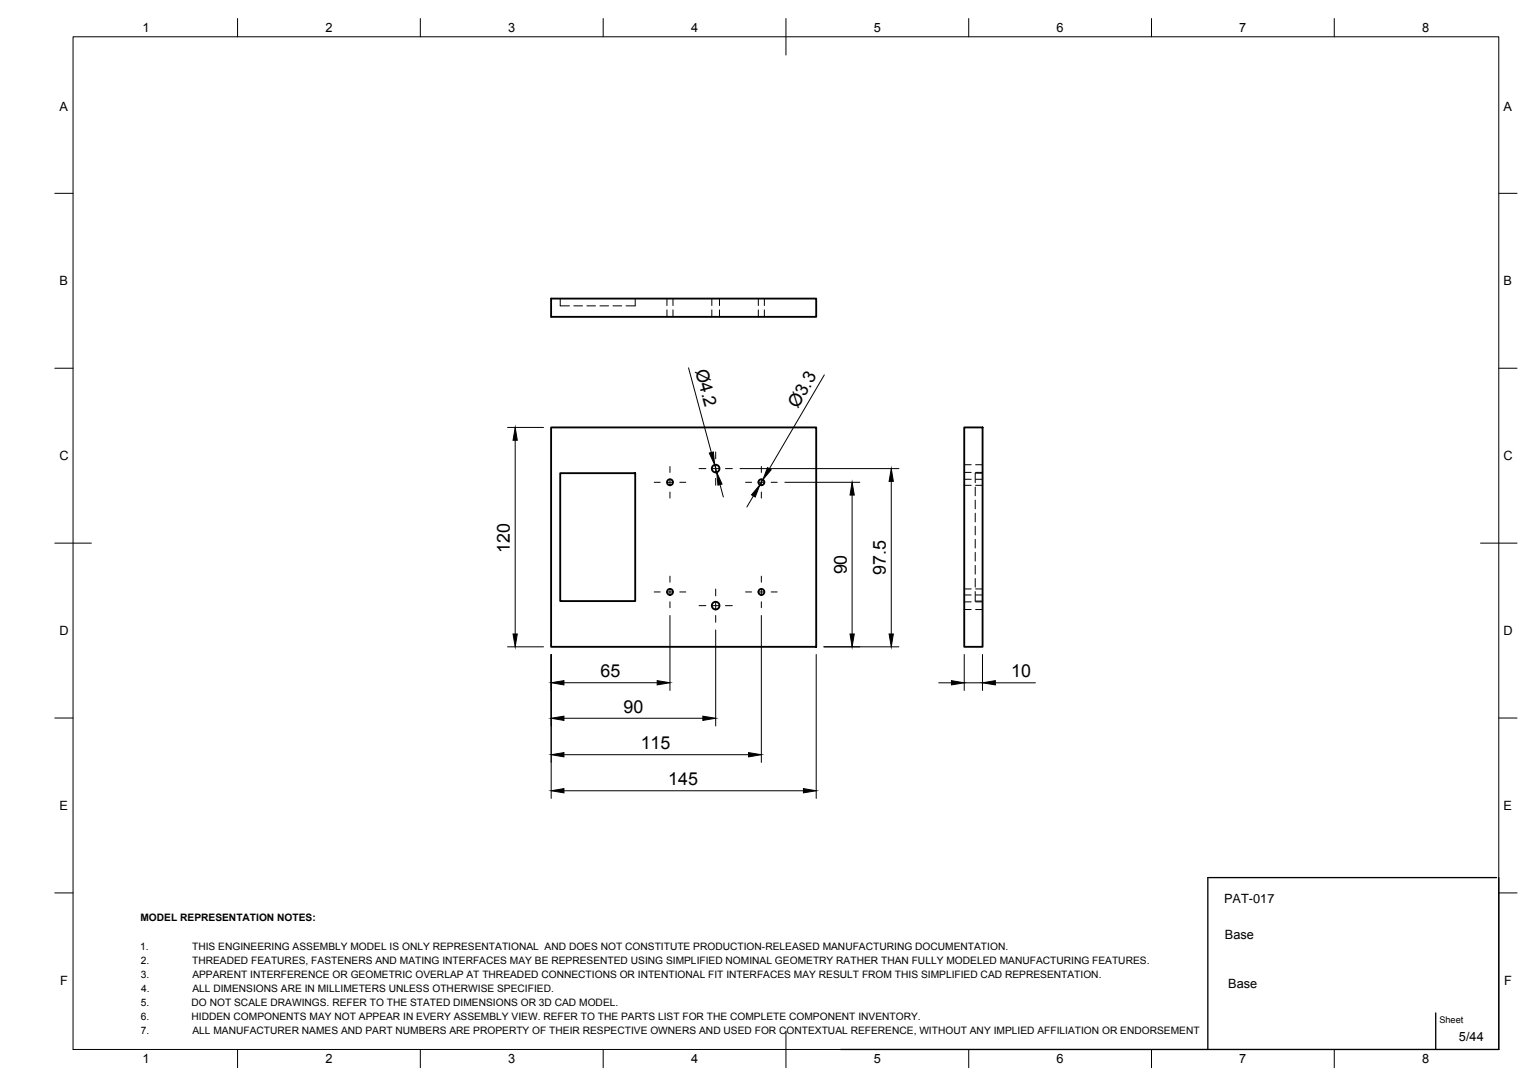
ISO-10303-21;
HEADER;
/* Generated by software containing ST-Developer
 * from STEP Tools, Inc. (www.steptools.com) 
 */

FILE_DESCRIPTION(
/* description */ ('Cam-and-follower valve demonstrator'),
/* implementation_level */ '2;1');

FILE_NAME(
/* name */ 'Base.step',
/* time_stamp */ '2026-10-28T03:25:17-07:00',
/* author */ (''),
/* organization */ (''),
/* preprocessor_version */ 'ST-DEVELOPER v20.2',
/* originating_system */ 'Autodesk Translation Framework v15.17.0.0',
/* authorisation */ '');

FILE_SCHEMA (('AUTOMOTIVE_DESIGN { 1 0 10303 214 3 1 1 }'));
ENDSEC;

DATA;
#10=MECHANICAL_DESIGN_GEOMETRIC_PRESENTATION_REPRESENTATION('',(#412),#12896);
#340=SHAPE_REPRESENTATION_RELATIONSHIP('SRR','None',#13056,#376);
#376=ADVANCED_BREP_SHAPE_REPRESENTATION('',(#455),#12856);
#412=STYLED_ITEM('',(#13309),#455);
#455=MANIFOLD_SOLID_BREP('Body1',#6179);
#495=FACE_BOUND('',#1479,.T.);
#496=FACE_BOUND('',#1480,.T.);
#497=FACE_BOUND('',#1481,.T.);
#498=FACE_BOUND('',#1482,.T.);
#499=FACE_BOUND('',#1483,.T.);
#500=FACE_BOUND('',#1484,.T.);
#501=FACE_BOUND('',#1485,.T.);
#502=FACE_BOUND('',#1487,.T.);
#503=FACE_BOUND('',#1488,.T.);
#504=FACE_BOUND('',#1489,.T.);
#505=FACE_BOUND('',#1490,.T.);
#506=FACE_BOUND('',#1491,.T.);
#507=FACE_BOUND('',#1492,.T.);
#659=CIRCLE('',#6631,0.21);
#660=CIRCLE('',#6632,0.21);
#661=CIRCLE('',#6634,0.21);
#662=CIRCLE('',#6635,0.21);
#663=CIRCLE('',#6637,0.165);
#664=CIRCLE('',#6638,0.165);
#665=CIRCLE('',#6640,0.165);
#666=CIRCLE('',#6641,0.165);
#667=CIRCLE('',#6643,0.165);
#668=CIRCLE('',#6644,0.165);
#669=CIRCLE('',#6646,0.165);
#670=CIRCLE('',#6647,0.165);
#973=CYLINDRICAL_SURFACE('',#6630,0.21);
#974=CYLINDRICAL_SURFACE('',#6633,0.21);
#975=CYLINDRICAL_SURFACE('',#6636,0.165);
#976=CYLINDRICAL_SURFACE('',#6639,0.165);
#977=CYLINDRICAL_SURFACE('',#6642,0.165);
#978=CYLINDRICAL_SURFACE('',#6645,0.165);
#1095=FACE_OUTER_BOUND('',#1463,.T.);
#1096=FACE_OUTER_BOUND('',#1464,.T.);
#1097=FACE_OUTER_BOUND('',#1465,.T.);
#1098=FACE_OUTER_BOUND('',#1466,.T.);
#1099=FACE_OUTER_BOUND('',#1467,.T.);
#1100=FACE_OUTER_BOUND('',#1468,.T.);
#1101=FACE_OUTER_BOUND('',#1469,.T.);
#1102=FACE_OUTER_BOUND('',#1470,.T.);
#1103=FACE_OUTER_BOUND('',#1471,.T.);
#1104=FACE_OUTER_BOUND('',#1472,.T.);
#1105=FACE_OUTER_BOUND('',#1473,.T.);
#1106=FACE_OUTER_BOUND('',#1474,.T.);
#1107=FACE_OUTER_BOUND('',#1475,.T.);
#1108=FACE_OUTER_BOUND('',#1476,.T.);
#1109=FACE_OUTER_BOUND('',#1477,.T.);
#1110=FACE_OUTER_BOUND('',#1478,.T.);
#1111=FACE_OUTER_BOUND('',#1486,.T.);
#1463=EDGE_LOOP('',(#4095,#4096,#4097,#4098));
#1464=EDGE_LOOP('',(#4099,#4100,#4101,#4102));
#1465=EDGE_LOOP('',(#4103,#4104,#4105,#4106));
#1466=EDGE_LOOP('',(#4107,#4108,#4109,#4110));
#1467=EDGE_LOOP('',(#4111,#4112,#4113,#4114));
#1468=EDGE_LOOP('',(#4115,#4116,#4117,#4118));
#1469=EDGE_LOOP('',(#4119,#4120,#4121,#4122));
#1470=EDGE_LOOP('',(#4123,#4124,#4125,#4126));
#1471=EDGE_LOOP('',(#4127,#4128,#4129,#4130));
#1472=EDGE_LOOP('',(#4131,#4132,#4133,#4134));
#1473=EDGE_LOOP('',(#4135,#4136,#4137,#4138));
#1474=EDGE_LOOP('',(#4139,#4140,#4141,#4142));
#1475=EDGE_LOOP('',(#4143,#4144,#4145,#4146));
#1476=EDGE_LOOP('',(#4147,#4148,#4149,#4150));
#1477=EDGE_LOOP('',(#4151,#4152,#4153,#4154));
#1478=EDGE_LOOP('',(#4155,#4156,#4157,#4158));
#1479=EDGE_LOOP('',(#4159,#4160,#4161,#4162));
#1480=EDGE_LOOP('',(#4163));
#1481=EDGE_LOOP('',(#4164));
#1482=EDGE_LOOP('',(#4165));
#1483=EDGE_LOOP('',(#4166));
#1484=EDGE_LOOP('',(#4167));
#1485=EDGE_LOOP('',(#4168));
#1486=EDGE_LOOP('',(#4169,#4170,#4171,#4172));
#1487=EDGE_LOOP('',(#4173));
#1488=EDGE_LOOP('',(#4174));
#1489=EDGE_LOOP('',(#4175));
#1490=EDGE_LOOP('',(#4176));
#1491=EDGE_LOOP('',(#4177));
#1492=EDGE_LOOP('',(#4178));
#1995=LINE('',#9426,#2417);
#1996=LINE('',#9428,#2418);
#1997=LINE('',#9430,#2419);
#1998=LINE('',#9431,#2420);
#1999=LINE('',#9434,#2421);
#2000=LINE('',#9436,#2422);
#2001=LINE('',#9437,#2423);
#2002=LINE('',#9440,#2424);
#2003=LINE('',#9442,#2425);
#2004=LINE('',#9443,#2426);
#2005=LINE('',#9445,#2427);
#2006=LINE('',#9446,#2428);
#2007=LINE('',#9452,#2429);
#2008=LINE('',#9458,#2430);
#2009=LINE('',#9464,#2431);
#2010=LINE('',#9470,#2432);
#2011=LINE('',#9476,#2433);
#2012=LINE('',#9482,#2434);
#2013=LINE('',#9487,#2435);
#2014=LINE('',#9489,#2436);
#2015=LINE('',#9491,#2437);
#2016=LINE('',#9492,#2438);
#2017=LINE('',#9495,#2439);
#2018=LINE('',#9497,#2440);
#2019=LINE('',#9498,#2441);
#2020=LINE('',#9501,#2442);
#2021=LINE('',#9503,#2443);
#2022=LINE('',#9504,#2444);
#2023=LINE('',#9506,#2445);
#2024=LINE('',#9507,#2446);
#2417=VECTOR('',#7422,1.);
#2418=VECTOR('',#7423,1.);
#2419=VECTOR('',#7424,1.);
#2420=VECTOR('',#7425,1.);
#2421=VECTOR('',#7428,1.);
#2422=VECTOR('',#7429,1.);
#2423=VECTOR('',#7430,1.);
#2424=VECTOR('',#7433,1.);
#2425=VECTOR('',#7434,1.);
#2426=VECTOR('',#7435,1.);
#2427=VECTOR('',#7438,1.);
#2428=VECTOR('',#7439,1.);
#2429=VECTOR('',#7446,0.21);
#2430=VECTOR('',#7453,0.21);
#2431=VECTOR('',#7460,0.165);
#2432=VECTOR('',#7467,0.165);
#2433=VECTOR('',#7474,0.165);
#2434=VECTOR('',#7481,0.165);
#2435=VECTOR('',#7486,1.);
#2436=VECTOR('',#7487,1.);
#2437=VECTOR('',#7488,1.);
#2438=VECTOR('',#7489,1.);
#2439=VECTOR('',#7492,1.);
#2440=VECTOR('',#7493,1.);
#2441=VECTOR('',#7494,1.);
#2442=VECTOR('',#7497,1.);
#2443=VECTOR('',#7498,1.);
#2444=VECTOR('',#7499,1.);
#2445=VECTOR('',#7502,1.);
#2446=VECTOR('',#7503,1.);
#2839=VERTEX_POINT('',#9424);
#2840=VERTEX_POINT('',#9425);
#2841=VERTEX_POINT('',#9427);
#2842=VERTEX_POINT('',#9429);
#2843=VERTEX_POINT('',#9433);
#2844=VERTEX_POINT('',#9435);
#2845=VERTEX_POINT('',#9439);
#2846=VERTEX_POINT('',#9441);
#2847=VERTEX_POINT('',#9449);
#2848=VERTEX_POINT('',#9451);
#2849=VERTEX_POINT('',#9455);
#2850=VERTEX_POINT('',#9457);
#2851=VERTEX_POINT('',#9461);
#2852=VERTEX_POINT('',#9463);
#2853=VERTEX_POINT('',#9467);
#2854=VERTEX_POINT('',#9469);
#2855=VERTEX_POINT('',#9473);
#2856=VERTEX_POINT('',#9475);
#2857=VERTEX_POINT('',#9479);
#2858=VERTEX_POINT('',#9481);
#2859=VERTEX_POINT('',#9485);
#2860=VERTEX_POINT('',#9486);
#2861=VERTEX_POINT('',#9488);
#2862=VERTEX_POINT('',#9490);
#2863=VERTEX_POINT('',#9494);
#2864=VERTEX_POINT('',#9496);
#2865=VERTEX_POINT('',#9500);
#2866=VERTEX_POINT('',#9502);
#3344=EDGE_CURVE('',#2839,#2840,#1995,.T.);
#3345=EDGE_CURVE('',#2841,#2839,#1996,.T.);
#3346=EDGE_CURVE('',#2842,#2841,#1997,.T.);
#3347=EDGE_CURVE('',#2842,#2840,#1998,.T.);
#3348=EDGE_CURVE('',#2840,#2843,#1999,.T.);
#3349=EDGE_CURVE('',#2844,#2842,#2000,.T.);
#3350=EDGE_CURVE('',#2844,#2843,#2001,.T.);
#3351=EDGE_CURVE('',#2843,#2845,#2002,.T.);
#3352=EDGE_CURVE('',#2846,#2844,#2003,.T.);
#3353=EDGE_CURVE('',#2846,#2845,#2004,.T.);
#3354=EDGE_CURVE('',#2845,#2839,#2005,.T.);
#3355=EDGE_CURVE('',#2841,#2846,#2006,.T.);
#3356=EDGE_CURVE('',#2847,#2847,#659,.T.);
#3357=EDGE_CURVE('',#2847,#2848,#2007,.T.);
#3358=EDGE_CURVE('',#2848,#2848,#660,.T.);
#3359=EDGE_CURVE('',#2849,#2849,#661,.T.);
#3360=EDGE_CURVE('',#2849,#2850,#2008,.T.);
#3361=EDGE_CURVE('',#2850,#2850,#662,.T.);
#3362=EDGE_CURVE('',#2851,#2851,#663,.T.);
#3363=EDGE_CURVE('',#2851,#2852,#2009,.T.);
#3364=EDGE_CURVE('',#2852,#2852,#664,.T.);
#3365=EDGE_CURVE('',#2853,#2853,#665,.T.);
#3366=EDGE_CURVE('',#2853,#2854,#2010,.T.);
#3367=EDGE_CURVE('',#2854,#2854,#666,.T.);
#3368=EDGE_CURVE('',#2855,#2855,#667,.T.);
#3369=EDGE_CURVE('',#2855,#2856,#2011,.T.);
#3370=EDGE_CURVE('',#2856,#2856,#668,.T.);
#3371=EDGE_CURVE('',#2857,#2857,#669,.T.);
#3372=EDGE_CURVE('',#2857,#2858,#2012,.T.);
#3373=EDGE_CURVE('',#2858,#2858,#670,.T.);
#3374=EDGE_CURVE('',#2859,#2860,#2013,.T.);
#3375=EDGE_CURVE('',#2860,#2861,#2014,.T.);
#3376=EDGE_CURVE('',#2862,#2861,#2015,.T.);
#3377=EDGE_CURVE('',#2859,#2862,#2016,.T.);
#3378=EDGE_CURVE('',#2863,#2859,#2017,.T.);
#3379=EDGE_CURVE('',#2864,#2862,#2018,.T.);
#3380=EDGE_CURVE('',#2863,#2864,#2019,.T.);
#3381=EDGE_CURVE('',#2865,#2863,#2020,.T.);
#3382=EDGE_CURVE('',#2866,#2864,#2021,.T.);
#3383=EDGE_CURVE('',#2865,#2866,#2022,.T.);
#3384=EDGE_CURVE('',#2860,#2865,#2023,.T.);
#3385=EDGE_CURVE('',#2861,#2866,#2024,.T.);
#4095=ORIENTED_EDGE('',*,*,#3344,.F.);
#4096=ORIENTED_EDGE('',*,*,#3345,.F.);
#4097=ORIENTED_EDGE('',*,*,#3346,.F.);
#4098=ORIENTED_EDGE('',*,*,#3347,.T.);
#4099=ORIENTED_EDGE('',*,*,#3348,.F.);
#4100=ORIENTED_EDGE('',*,*,#3347,.F.);
#4101=ORIENTED_EDGE('',*,*,#3349,.F.);
#4102=ORIENTED_EDGE('',*,*,#3350,.T.);
#4103=ORIENTED_EDGE('',*,*,#3351,.F.);
#4104=ORIENTED_EDGE('',*,*,#3350,.F.);
#4105=ORIENTED_EDGE('',*,*,#3352,.F.);
#4106=ORIENTED_EDGE('',*,*,#3353,.T.);
#4107=ORIENTED_EDGE('',*,*,#3354,.F.);
#4108=ORIENTED_EDGE('',*,*,#3353,.F.);
#4109=ORIENTED_EDGE('',*,*,#3355,.F.);
#4110=ORIENTED_EDGE('',*,*,#3345,.T.);
#4111=ORIENTED_EDGE('',*,*,#3349,.T.);
#4112=ORIENTED_EDGE('',*,*,#3346,.T.);
#4113=ORIENTED_EDGE('',*,*,#3355,.T.);
#4114=ORIENTED_EDGE('',*,*,#3352,.T.);
#4115=ORIENTED_EDGE('',*,*,#3356,.F.);
#4116=ORIENTED_EDGE('',*,*,#3357,.T.);
#4117=ORIENTED_EDGE('',*,*,#3358,.F.);
#4118=ORIENTED_EDGE('',*,*,#3357,.F.);
#4119=ORIENTED_EDGE('',*,*,#3359,.F.);
#4120=ORIENTED_EDGE('',*,*,#3360,.T.);
#4121=ORIENTED_EDGE('',*,*,#3361,.F.);
#4122=ORIENTED_EDGE('',*,*,#3360,.F.);
#4123=ORIENTED_EDGE('',*,*,#3362,.F.);
#4124=ORIENTED_EDGE('',*,*,#3363,.T.);
#4125=ORIENTED_EDGE('',*,*,#3364,.F.);
#4126=ORIENTED_EDGE('',*,*,#3363,.F.);
#4127=ORIENTED_EDGE('',*,*,#3365,.F.);
#4128=ORIENTED_EDGE('',*,*,#3366,.T.);
#4129=ORIENTED_EDGE('',*,*,#3367,.F.);
#4130=ORIENTED_EDGE('',*,*,#3366,.F.);
#4131=ORIENTED_EDGE('',*,*,#3368,.F.);
#4132=ORIENTED_EDGE('',*,*,#3369,.T.);
#4133=ORIENTED_EDGE('',*,*,#3370,.F.);
#4134=ORIENTED_EDGE('',*,*,#3369,.F.);
#4135=ORIENTED_EDGE('',*,*,#3371,.F.);
#4136=ORIENTED_EDGE('',*,*,#3372,.T.);
#4137=ORIENTED_EDGE('',*,*,#3373,.F.);
#4138=ORIENTED_EDGE('',*,*,#3372,.F.);
#4139=ORIENTED_EDGE('',*,*,#3374,.T.);
#4140=ORIENTED_EDGE('',*,*,#3375,.T.);
#4141=ORIENTED_EDGE('',*,*,#3376,.F.);
#4142=ORIENTED_EDGE('',*,*,#3377,.F.);
#4143=ORIENTED_EDGE('',*,*,#3378,.T.);
#4144=ORIENTED_EDGE('',*,*,#3377,.T.);
#4145=ORIENTED_EDGE('',*,*,#3379,.F.);
#4146=ORIENTED_EDGE('',*,*,#3380,.F.);
#4147=ORIENTED_EDGE('',*,*,#3381,.T.);
#4148=ORIENTED_EDGE('',*,*,#3380,.T.);
#4149=ORIENTED_EDGE('',*,*,#3382,.F.);
#4150=ORIENTED_EDGE('',*,*,#3383,.F.);
#4151=ORIENTED_EDGE('',*,*,#3384,.T.);
#4152=ORIENTED_EDGE('',*,*,#3383,.T.);
#4153=ORIENTED_EDGE('',*,*,#3385,.F.);
#4154=ORIENTED_EDGE('',*,*,#3375,.F.);
#4155=ORIENTED_EDGE('',*,*,#3385,.T.);
#4156=ORIENTED_EDGE('',*,*,#3382,.T.);
#4157=ORIENTED_EDGE('',*,*,#3379,.T.);
#4158=ORIENTED_EDGE('',*,*,#3376,.T.);
#4159=ORIENTED_EDGE('',*,*,#3351,.T.);
#4160=ORIENTED_EDGE('',*,*,#3354,.T.);
#4161=ORIENTED_EDGE('',*,*,#3344,.T.);
#4162=ORIENTED_EDGE('',*,*,#3348,.T.);
#4163=ORIENTED_EDGE('',*,*,#3358,.T.);
#4164=ORIENTED_EDGE('',*,*,#3361,.T.);
#4165=ORIENTED_EDGE('',*,*,#3364,.T.);
#4166=ORIENTED_EDGE('',*,*,#3367,.T.);
#4167=ORIENTED_EDGE('',*,*,#3370,.T.);
#4168=ORIENTED_EDGE('',*,*,#3373,.T.);
#4169=ORIENTED_EDGE('',*,*,#3384,.F.);
#4170=ORIENTED_EDGE('',*,*,#3374,.F.);
#4171=ORIENTED_EDGE('',*,*,#3378,.F.);
#4172=ORIENTED_EDGE('',*,*,#3381,.F.);
#4173=ORIENTED_EDGE('',*,*,#3356,.T.);
#4174=ORIENTED_EDGE('',*,*,#3359,.T.);
#4175=ORIENTED_EDGE('',*,*,#3362,.T.);
#4176=ORIENTED_EDGE('',*,*,#3365,.T.);
#4177=ORIENTED_EDGE('',*,*,#3368,.T.);
#4178=ORIENTED_EDGE('',*,*,#3371,.T.);
#5597=PLANE('',#6625);
#5598=PLANE('',#6626);
#5599=PLANE('',#6627);
#5600=PLANE('',#6628);
#5601=PLANE('',#6629);
#5602=PLANE('',#6648);
#5603=PLANE('',#6649);
#5604=PLANE('',#6650);
#5605=PLANE('',#6651);
#5606=PLANE('',#6652);
#5607=PLANE('',#6653);
#5811=ADVANCED_FACE('',(#1095),#5597,.F.);
#5812=ADVANCED_FACE('',(#1096),#5598,.F.);
#5813=ADVANCED_FACE('',(#1097),#5599,.F.);
#5814=ADVANCED_FACE('',(#1098),#5600,.F.);
#5815=ADVANCED_FACE('',(#1099),#5601,.T.);
#5816=ADVANCED_FACE('',(#1100),#973,.F.);
#5817=ADVANCED_FACE('',(#1101),#974,.F.);
#5818=ADVANCED_FACE('',(#1102),#975,.F.);
#5819=ADVANCED_FACE('',(#1103),#976,.F.);
#5820=ADVANCED_FACE('',(#1104),#977,.F.);
#5821=ADVANCED_FACE('',(#1105),#978,.F.);
#5822=ADVANCED_FACE('',(#1106),#5602,.T.);
#5823=ADVANCED_FACE('',(#1107),#5603,.T.);
#5824=ADVANCED_FACE('',(#1108),#5604,.T.);
#5825=ADVANCED_FACE('',(#1109),#5605,.T.);
#5826=ADVANCED_FACE('',(#1110,#495,#496,#497,#498,#499,#500,#501),#5606,
 .T.);
#5827=ADVANCED_FACE('',(#1111,#502,#503,#504,#505,#506,#507),#5607,.F.);
#6179=CLOSED_SHELL('',(#5811,#5812,#5813,#5814,#5815,#5816,#5817,#5818,
#5819,#5820,#5821,#5822,#5823,#5824,#5825,#5826,#5827));
#6624=AXIS2_PLACEMENT_3D('',#9422,#7418,#7419);
#6625=AXIS2_PLACEMENT_3D('',#9423,#7420,#7421);
#6626=AXIS2_PLACEMENT_3D('',#9432,#7426,#7427);
#6627=AXIS2_PLACEMENT_3D('',#9438,#7431,#7432);
#6628=AXIS2_PLACEMENT_3D('',#9444,#7436,#7437);
#6629=AXIS2_PLACEMENT_3D('',#9447,#7440,#7441);
#6630=AXIS2_PLACEMENT_3D('',#9448,#7442,#7443);
#6631=AXIS2_PLACEMENT_3D('',#9450,#7444,#7445);
#6632=AXIS2_PLACEMENT_3D('',#9453,#7447,#7448);
#6633=AXIS2_PLACEMENT_3D('',#9454,#7449,#7450);
#6634=AXIS2_PLACEMENT_3D('',#9456,#7451,#7452);
#6635=AXIS2_PLACEMENT_3D('',#9459,#7454,#7455);
#6636=AXIS2_PLACEMENT_3D('',#9460,#7456,#7457);
#6637=AXIS2_PLACEMENT_3D('',#9462,#7458,#7459);
#6638=AXIS2_PLACEMENT_3D('',#9465,#7461,#7462);
#6639=AXIS2_PLACEMENT_3D('',#9466,#7463,#7464);
#6640=AXIS2_PLACEMENT_3D('',#9468,#7465,#7466);
#6641=AXIS2_PLACEMENT_3D('',#9471,#7468,#7469);
#6642=AXIS2_PLACEMENT_3D('',#9472,#7470,#7471);
#6643=AXIS2_PLACEMENT_3D('',#9474,#7472,#7473);
#6644=AXIS2_PLACEMENT_3D('',#9477,#7475,#7476);
#6645=AXIS2_PLACEMENT_3D('',#9478,#7477,#7478);
#6646=AXIS2_PLACEMENT_3D('',#9480,#7479,#7480);
#6647=AXIS2_PLACEMENT_3D('',#9483,#7482,#7483);
#6648=AXIS2_PLACEMENT_3D('',#9484,#7484,#7485);
#6649=AXIS2_PLACEMENT_3D('',#9493,#7490,#7491);
#6650=AXIS2_PLACEMENT_3D('',#9499,#7495,#7496);
#6651=AXIS2_PLACEMENT_3D('',#9505,#7500,#7501);
#6652=AXIS2_PLACEMENT_3D('',#9508,#7504,#7505);
#6653=AXIS2_PLACEMENT_3D('',#9509,#7506,#7507);
#7418=DIRECTION('axis',(0.,0.,1.));
#7419=DIRECTION('refdir',(1.,0.,0.));
#7420=DIRECTION('center_axis',(0.,-1.,0.));
#7421=DIRECTION('ref_axis',(1.,0.,0.));
#7422=DIRECTION('',(-1.,0.,0.));
#7423=DIRECTION('',(0.,0.,1.));
#7424=DIRECTION('',(1.,0.,0.));
#7425=DIRECTION('',(0.,0.,1.));
#7426=DIRECTION('center_axis',(-1.,0.,0.));
#7427=DIRECTION('ref_axis',(0.,-1.,0.));
#7428=DIRECTION('',(0.,1.,0.));
#7429=DIRECTION('',(0.,-1.,0.));
#7430=DIRECTION('',(0.,0.,1.));
#7431=DIRECTION('center_axis',(0.,1.,0.));
#7432=DIRECTION('ref_axis',(-1.,0.,0.));
#7433=DIRECTION('',(1.,0.,0.));
#7434=DIRECTION('',(-1.,0.,0.));
#7435=DIRECTION('',(0.,0.,1.));
#7436=DIRECTION('center_axis',(1.,0.,0.));
#7437=DIRECTION('ref_axis',(0.,1.,0.));
#7438=DIRECTION('',(0.,-1.,0.));
#7439=DIRECTION('',(0.,1.,0.));
#7440=DIRECTION('center_axis',(0.,0.,1.));
#7441=DIRECTION('ref_axis',(1.,0.,0.));
#7442=DIRECTION('center_axis',(0.,0.,1.));
#7443=DIRECTION('ref_axis',(1.,0.,0.));
#7444=DIRECTION('center_axis',(0.,0.,1.));
#7445=DIRECTION('ref_axis',(1.,0.,0.));
#7446=DIRECTION('',(0.,0.,1.));
#7447=DIRECTION('center_axis',(0.,0.,-1.));
#7448=DIRECTION('ref_axis',(1.,0.,0.));
#7449=DIRECTION('center_axis',(0.,0.,1.));
#7450=DIRECTION('ref_axis',(1.,0.,0.));
#7451=DIRECTION('center_axis',(0.,0.,1.));
#7452=DIRECTION('ref_axis',(1.,0.,0.));
#7453=DIRECTION('',(0.,0.,1.));
#7454=DIRECTION('center_axis',(0.,0.,-1.));
#7455=DIRECTION('ref_axis',(1.,0.,0.));
#7456=DIRECTION('center_axis',(0.,0.,1.));
#7457=DIRECTION('ref_axis',(1.,0.,0.));
#7458=DIRECTION('center_axis',(0.,0.,1.));
#7459=DIRECTION('ref_axis',(1.,0.,0.));
#7460=DIRECTION('',(0.,0.,1.));
#7461=DIRECTION('center_axis',(0.,0.,-1.));
#7462=DIRECTION('ref_axis',(1.,0.,0.));
#7463=DIRECTION('center_axis',(0.,0.,1.));
#7464=DIRECTION('ref_axis',(1.,0.,0.));
#7465=DIRECTION('center_axis',(0.,0.,1.));
#7466=DIRECTION('ref_axis',(1.,0.,0.));
#7467=DIRECTION('',(0.,0.,1.));
#7468=DIRECTION('center_axis',(0.,0.,-1.));
#7469=DIRECTION('ref_axis',(1.,0.,0.));
#7470=DIRECTION('center_axis',(0.,0.,1.));
#7471=DIRECTION('ref_axis',(1.,0.,0.));
#7472=DIRECTION('center_axis',(0.,0.,1.));
#7473=DIRECTION('ref_axis',(1.,0.,0.));
#7474=DIRECTION('',(0.,0.,1.));
#7475=DIRECTION('center_axis',(0.,0.,-1.));
#7476=DIRECTION('ref_axis',(1.,0.,0.));
#7477=DIRECTION('center_axis',(0.,0.,1.));
#7478=DIRECTION('ref_axis',(1.,0.,0.));
#7479=DIRECTION('center_axis',(0.,0.,1.));
#7480=DIRECTION('ref_axis',(1.,0.,0.));
#7481=DIRECTION('',(0.,0.,1.));
#7482=DIRECTION('center_axis',(0.,0.,-1.));
#7483=DIRECTION('ref_axis',(1.,0.,0.));
#7484=DIRECTION('center_axis',(0.,1.,0.));
#7485=DIRECTION('ref_axis',(-1.,0.,0.));
#7486=DIRECTION('',(-1.,0.,0.));
#7487=DIRECTION('',(0.,0.,1.));
#7488=DIRECTION('',(-1.,0.,0.));
#7489=DIRECTION('',(0.,0.,1.));
#7490=DIRECTION('center_axis',(1.,0.,0.));
#7491=DIRECTION('ref_axis',(0.,1.,0.));
#7492=DIRECTION('',(0.,1.,0.));
#7493=DIRECTION('',(0.,1.,0.));
#7494=DIRECTION('',(0.,0.,1.));
#7495=DIRECTION('center_axis',(0.,-1.,0.));
#7496=DIRECTION('ref_axis',(1.,0.,0.));
#7497=DIRECTION('',(1.,0.,0.));
#7498=DIRECTION('',(1.,0.,0.));
#7499=DIRECTION('',(0.,0.,1.));
#7500=DIRECTION('center_axis',(-1.,0.,0.));
#7501=DIRECTION('ref_axis',(0.,-1.,0.));
#7502=DIRECTION('',(0.,-1.,0.));
#7503=DIRECTION('',(0.,-1.,0.));
#7504=DIRECTION('center_axis',(0.,0.,1.));
#7505=DIRECTION('ref_axis',(1.,0.,0.));
#7506=DIRECTION('center_axis',(0.,0.,1.));
#7507=DIRECTION('ref_axis',(1.,0.,0.));
#9422=CARTESIAN_POINT('',(0.,0.,0.));
#9423=CARTESIAN_POINT('Origin',(-3.5,4.4,0.6));
#9424=CARTESIAN_POINT('',(3.5,4.4,1.));
#9425=CARTESIAN_POINT('',(-3.5,4.4,1.));
#9426=CARTESIAN_POINT('',(-1.75,4.4,1.));
#9427=CARTESIAN_POINT('',(3.5,4.4,0.6));
#9428=CARTESIAN_POINT('',(3.5,4.4,0.6));
#9429=CARTESIAN_POINT('',(-3.5,4.4,0.6));
#9430=CARTESIAN_POINT('',(-3.5,4.4,0.6));
#9431=CARTESIAN_POINT('',(-3.5,4.4,0.6));
#9432=CARTESIAN_POINT('Origin',(-3.5,8.5,0.6));
#9433=CARTESIAN_POINT('',(-3.5,8.5,1.));
#9434=CARTESIAN_POINT('',(-3.5,5.125,1.));
#9435=CARTESIAN_POINT('',(-3.5,8.5,0.6));
#9436=CARTESIAN_POINT('',(-3.5,8.5,0.6));
#9437=CARTESIAN_POINT('',(-3.5,8.5,0.6));
#9438=CARTESIAN_POINT('Origin',(3.5,8.5,0.6));
#9439=CARTESIAN_POINT('',(3.5,8.5,1.));
#9440=CARTESIAN_POINT('',(1.75,8.5,1.));
#9441=CARTESIAN_POINT('',(3.5,8.5,0.6));
#9442=CARTESIAN_POINT('',(3.5,8.5,0.6));
#9443=CARTESIAN_POINT('',(3.5,8.5,0.6));
#9444=CARTESIAN_POINT('Origin',(3.5,4.4,0.6));
#9445=CARTESIAN_POINT('',(3.5,3.075,1.));
#9446=CARTESIAN_POINT('',(3.5,4.4,0.6));
#9447=CARTESIAN_POINT('Origin',(0.,6.45,0.6));
#9448=CARTESIAN_POINT('Origin',(3.75,0.,-0.1));
#9449=CARTESIAN_POINT('',(3.54,-2.57175827820944E-17,0.));
#9450=CARTESIAN_POINT('Origin',(3.75,0.,0.));
#9451=CARTESIAN_POINT('',(3.54,2.57175827820944E-17,1.));
#9452=CARTESIAN_POINT('',(3.54,-2.57175827820944E-17,-0.1));
#9453=CARTESIAN_POINT('Origin',(3.75,0.,1.));
#9454=CARTESIAN_POINT('Origin',(-3.75,0.,-0.1));
#9455=CARTESIAN_POINT('',(-3.96,-2.57175827820944E-17,0.));
#9456=CARTESIAN_POINT('Origin',(-3.75,0.,0.));
#9457=CARTESIAN_POINT('',(-3.96,2.57175827820944E-17,1.));
#9458=CARTESIAN_POINT('',(-3.96,-2.57175827820944E-17,-0.1));
#9459=CARTESIAN_POINT('Origin',(-3.75,0.,1.));
#9460=CARTESIAN_POINT('Origin',(-3.,2.5,-0.1));
#9461=CARTESIAN_POINT('',(-3.165,2.5,0.));
#9462=CARTESIAN_POINT('Origin',(-3.,2.5,0.));
#9463=CARTESIAN_POINT('',(-3.165,2.5,1.));
#9464=CARTESIAN_POINT('',(-3.165,2.5,-0.1));
#9465=CARTESIAN_POINT('Origin',(-3.,2.5,1.));
#9466=CARTESIAN_POINT('Origin',(3.,2.5,-0.1));
#9467=CARTESIAN_POINT('',(2.835,2.5,0.));
#9468=CARTESIAN_POINT('Origin',(3.,2.5,0.));
#9469=CARTESIAN_POINT('',(2.835,2.5,1.));
#9470=CARTESIAN_POINT('',(2.835,2.5,-0.1));
#9471=CARTESIAN_POINT('Origin',(3.,2.5,1.));
#9472=CARTESIAN_POINT('Origin',(-3.,-2.5,-0.1));
#9473=CARTESIAN_POINT('',(-3.165,-2.5,0.));
#9474=CARTESIAN_POINT('Origin',(-3.,-2.5,0.));
#9475=CARTESIAN_POINT('',(-3.165,-2.5,1.));
#9476=CARTESIAN_POINT('',(-3.165,-2.5,-0.1));
#9477=CARTESIAN_POINT('Origin',(-3.,-2.5,1.));
#9478=CARTESIAN_POINT('Origin',(3.,-2.5,-0.1));
#9479=CARTESIAN_POINT('',(2.835,-2.5,0.));
#9480=CARTESIAN_POINT('Origin',(3.,-2.5,0.));
#9481=CARTESIAN_POINT('',(2.835,-2.5,1.));
#9482=CARTESIAN_POINT('',(2.835,-2.5,-0.1));
#9483=CARTESIAN_POINT('Origin',(3.,-2.5,1.));
#9484=CARTESIAN_POINT('Origin',(6.,9.,0.));
#9485=CARTESIAN_POINT('',(6.,9.,0.));
#9486=CARTESIAN_POINT('',(-6.,9.,0.));
#9487=CARTESIAN_POINT('',(6.,9.,0.));
#9488=CARTESIAN_POINT('',(-6.,9.,1.));
#9489=CARTESIAN_POINT('',(-6.,9.,0.));
#9490=CARTESIAN_POINT('',(6.,9.,1.));
#9491=CARTESIAN_POINT('',(6.,9.,1.));
#9492=CARTESIAN_POINT('',(6.,9.,0.));
#9493=CARTESIAN_POINT('Origin',(6.,-5.5,0.));
#9494=CARTESIAN_POINT('',(6.,-5.5,0.));
#9495=CARTESIAN_POINT('',(6.,-5.5,0.));
#9496=CARTESIAN_POINT('',(6.,-5.5,1.));
#9497=CARTESIAN_POINT('',(6.,-5.5,1.));
#9498=CARTESIAN_POINT('',(6.,-5.5,0.));
#9499=CARTESIAN_POINT('Origin',(-6.,-5.5,0.));
#9500=CARTESIAN_POINT('',(-6.,-5.5,0.));
#9501=CARTESIAN_POINT('',(-6.,-5.5,0.));
#9502=CARTESIAN_POINT('',(-6.,-5.5,1.));
#9503=CARTESIAN_POINT('',(-6.,-5.5,1.));
#9504=CARTESIAN_POINT('',(-6.,-5.5,0.));
#9505=CARTESIAN_POINT('Origin',(-6.,9.,0.));
#9506=CARTESIAN_POINT('',(-6.,9.,0.));
#9507=CARTESIAN_POINT('',(-6.,9.,1.));
#9508=CARTESIAN_POINT('Origin',(0.,1.75,1.));
#9509=CARTESIAN_POINT('Origin',(0.,1.75,0.));
#12813=UNCERTAINTY_MEASURE_WITH_UNIT(LENGTH_MEASURE(0.001),#12897,
'DISTANCE_ACCURACY_VALUE',
'Maximum model space distance between geometric entities at asserted c
onnectivities');
#12853=UNCERTAINTY_MEASURE_WITH_UNIT(LENGTH_MEASURE(0.001),#12897,
'DISTANCE_ACCURACY_VALUE',
'Maximum model space distance between geometric entities at asserted c
onnectivities');
#12856=(
GEOMETRIC_REPRESENTATION_CONTEXT(3)
GLOBAL_UNCERTAINTY_ASSIGNED_CONTEXT((#12813))
GLOBAL_UNIT_ASSIGNED_CONTEXT((#12897,#12899,#12900))
REPRESENTATION_CONTEXT('','3D')
);
#12896=(
GEOMETRIC_REPRESENTATION_CONTEXT(3)
GLOBAL_UNCERTAINTY_ASSIGNED_CONTEXT((#12853))
GLOBAL_UNIT_ASSIGNED_CONTEXT((#12897,#12899,#12900))
REPRESENTATION_CONTEXT('','3D')
);
#12897=(
LENGTH_UNIT()
NAMED_UNIT(*)
SI_UNIT(.CENTI.,.METRE.)
);
#12899=(
NAMED_UNIT(*)
PLANE_ANGLE_UNIT()
SI_UNIT($,.RADIAN.)
);
#12900=(
NAMED_UNIT(*)
SI_UNIT($,.STERADIAN.)
SOLID_ANGLE_UNIT()
);
#12903=SHAPE_DEFINITION_REPRESENTATION(#12945,#13056);
#12945=PRODUCT_DEFINITION_SHAPE('',$,#13099);
#13056=SHAPE_REPRESENTATION('',(#6624),#12856);
#13096=PRODUCT_DEFINITION_CONTEXT('part definition',#13224,'design');
#13099=PRODUCT_DEFINITION('Base','Base',#13141,#13096);
#13141=PRODUCT_DEFINITION_FORMATION('',$,#13228);
#13224=APPLICATION_CONTEXT(
'Core Data for Automotive Mechanical Design Process');
#13225=PRODUCT_CONTEXT('part definition',#13224,'mechanical');
#13228=PRODUCT('Base','Base','Base',(#13225));
#13303=COLOUR_RGB('Dark Blue',0.08,0.2,0.34);
#13304=FILL_AREA_STYLE_COLOUR('',#13303);
#13305=FILL_AREA_STYLE('',(#13304));
#13306=SURFACE_STYLE_FILL_AREA(#13305);
#13307=SURFACE_SIDE_STYLE('',(#13306));
#13308=SURFACE_STYLE_USAGE(.BOTH.,#13307);
#13309=PRESENTATION_STYLE_ASSIGNMENT((#13308));
ENDSEC;
END-ISO-10303-21;
